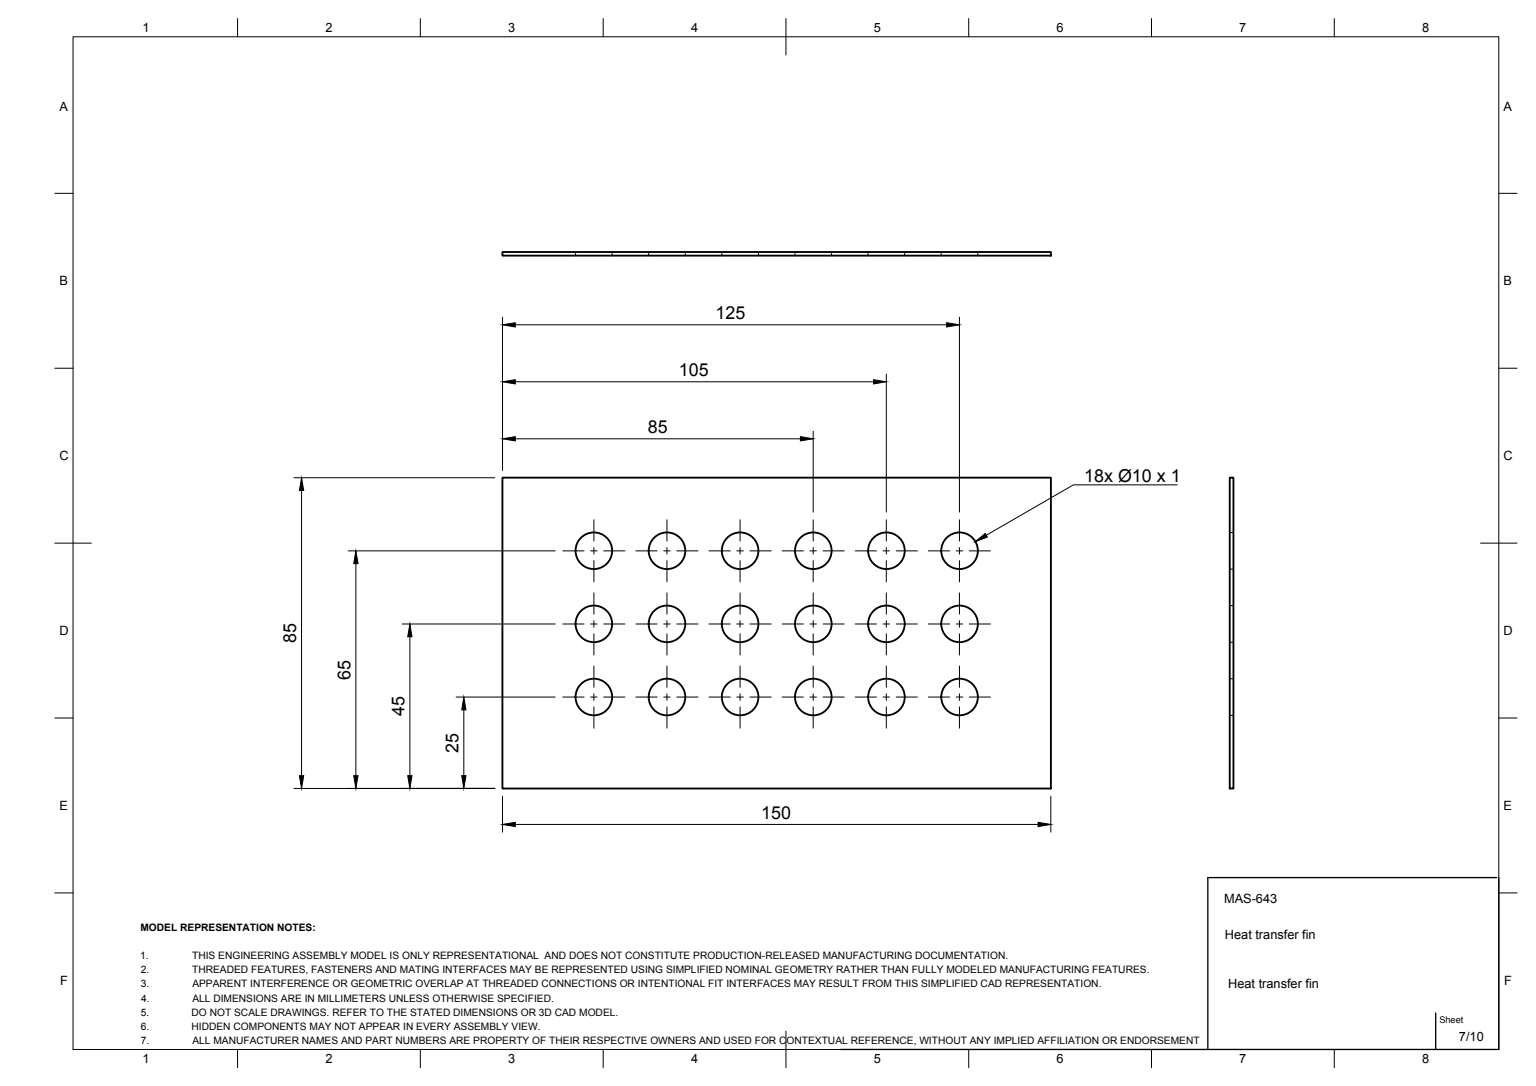
ISO-10303-21;
HEADER;
/* Generated by software containing ST-Developer
 * from STEP Tools, Inc. (www.steptools.com) 
 */

FILE_DESCRIPTION(
/* description */ ('Independent eighteen-tube parallel-flow evaporator geometry. Repeated
 machined headers and gasketed service covers, eighteen copper tubes, 
twenty-nine punched fins, threaded hose connections and bolted mountin
g feet. Native editable features and instanced parts. Braze details, w
orking fluid, pressure and thermal ratings require engineering selecti
on.'),
/* implementation_level */ '2;1');

FILE_NAME(
/* name */ 'Heat transfer fin.step',
/* time_stamp */ '2026-11-08T20:53:59-08:00',
/* author */ (''),
/* organization */ (''),
/* preprocessor_version */ 'ST-DEVELOPER v20.2',
/* originating_system */ 'Autodesk Translation Framework v15.17.0.0',
/* authorisation */ '');

FILE_SCHEMA (('AUTOMOTIVE_DESIGN { 1 0 10303 214 3 1 1 }'));
ENDSEC;

DATA;
#10=MECHANICAL_DESIGN_GEOMETRIC_PRESENTATION_REPRESENTATION('',(#337),#42620);
#317=SHAPE_REPRESENTATION_RELATIONSHIP('SRR','None',#42727,#327);
#327=ADVANCED_BREP_SHAPE_REPRESENTATION('',(#347),#42614);
#337=STYLED_ITEM('',(#42786),#347);
#347=MANIFOLD_SOLID_BREP('Body1',#10387);
#421=FACE_BOUND('',#1613,.T.);
#422=FACE_BOUND('',#1614,.T.);
#423=FACE_BOUND('',#1615,.T.);
#424=FACE_BOUND('',#1616,.T.);
#425=FACE_BOUND('',#1617,.T.);
#426=FACE_BOUND('',#1618,.T.);
#427=FACE_BOUND('',#1619,.T.);
#428=FACE_BOUND('',#1620,.T.);
#429=FACE_BOUND('',#1621,.T.);
#430=FACE_BOUND('',#1622,.T.);
#431=FACE_BOUND('',#1623,.T.);
#432=FACE_BOUND('',#1624,.T.);
#433=FACE_BOUND('',#1625,.T.);
#434=FACE_BOUND('',#1626,.T.);
#435=FACE_BOUND('',#1627,.T.);
#436=FACE_BOUND('',#1628,.T.);
#437=FACE_BOUND('',#1629,.T.);
#438=FACE_BOUND('',#1630,.T.);
#439=FACE_BOUND('',#1632,.T.);
#440=FACE_BOUND('',#1633,.T.);
#441=FACE_BOUND('',#1634,.T.);
#442=FACE_BOUND('',#1635,.T.);
#443=FACE_BOUND('',#1636,.T.);
#444=FACE_BOUND('',#1637,.T.);
#445=FACE_BOUND('',#1638,.T.);
#446=FACE_BOUND('',#1639,.T.);
#447=FACE_BOUND('',#1640,.T.);
#448=FACE_BOUND('',#1641,.T.);
#449=FACE_BOUND('',#1642,.T.);
#450=FACE_BOUND('',#1643,.T.);
#451=FACE_BOUND('',#1644,.T.);
#452=FACE_BOUND('',#1645,.T.);
#453=FACE_BOUND('',#1646,.T.);
#454=FACE_BOUND('',#1647,.T.);
#455=FACE_BOUND('',#1648,.T.);
#456=FACE_BOUND('',#1649,.T.);
#535=PLANE('',#11027);
#536=PLANE('',#11028);
#537=PLANE('',#11029);
#538=PLANE('',#11030);
#539=PLANE('',#11031);
#540=PLANE('',#11032);
#978=FACE_OUTER_BOUND('',#1590,.T.);
#979=FACE_OUTER_BOUND('',#1591,.T.);
#980=FACE_OUTER_BOUND('',#1592,.T.);
#981=FACE_OUTER_BOUND('',#1593,.T.);
#982=FACE_OUTER_BOUND('',#1594,.T.);
#983=FACE_OUTER_BOUND('',#1595,.T.);
#984=FACE_OUTER_BOUND('',#1596,.T.);
#985=FACE_OUTER_BOUND('',#1597,.T.);
#986=FACE_OUTER_BOUND('',#1598,.T.);
#987=FACE_OUTER_BOUND('',#1599,.T.);
#988=FACE_OUTER_BOUND('',#1600,.T.);
#989=FACE_OUTER_BOUND('',#1601,.T.);
#990=FACE_OUTER_BOUND('',#1602,.T.);
#991=FACE_OUTER_BOUND('',#1603,.T.);
#992=FACE_OUTER_BOUND('',#1604,.T.);
#993=FACE_OUTER_BOUND('',#1605,.T.);
#994=FACE_OUTER_BOUND('',#1606,.T.);
#995=FACE_OUTER_BOUND('',#1607,.T.);
#996=FACE_OUTER_BOUND('',#1608,.T.);
#997=FACE_OUTER_BOUND('',#1609,.T.);
#998=FACE_OUTER_BOUND('',#1610,.T.);
#999=FACE_OUTER_BOUND('',#1611,.T.);
#1000=FACE_OUTER_BOUND('',#1612,.T.);
#1001=FACE_OUTER_BOUND('',#1631,.T.);
#1590=EDGE_LOOP('',(#8543,#8544,#8545,#8546));
#1591=EDGE_LOOP('',(#8547,#8548,#8549,#8550));
#1592=EDGE_LOOP('',(#8551,#8552,#8553,#8554));
#1593=EDGE_LOOP('',(#8555,#8556,#8557,#8558));
#1594=EDGE_LOOP('',(#8559,#8560,#8561,#8562));
#1595=EDGE_LOOP('',(#8563,#8564,#8565,#8566));
#1596=EDGE_LOOP('',(#8567,#8568,#8569,#8570));
#1597=EDGE_LOOP('',(#8571,#8572,#8573,#8574));
#1598=EDGE_LOOP('',(#8575,#8576,#8577,#8578));
#1599=EDGE_LOOP('',(#8579,#8580,#8581,#8582));
#1600=EDGE_LOOP('',(#8583,#8584,#8585,#8586));
#1601=EDGE_LOOP('',(#8587,#8588,#8589,#8590));
#1602=EDGE_LOOP('',(#8591,#8592,#8593,#8594));
#1603=EDGE_LOOP('',(#8595,#8596,#8597,#8598));
#1604=EDGE_LOOP('',(#8599,#8600,#8601,#8602));
#1605=EDGE_LOOP('',(#8603,#8604,#8605,#8606));
#1606=EDGE_LOOP('',(#8607,#8608,#8609,#8610));
#1607=EDGE_LOOP('',(#8611,#8612,#8613,#8614));
#1608=EDGE_LOOP('',(#8615,#8616,#8617,#8618));
#1609=EDGE_LOOP('',(#8619,#8620,#8621,#8622));
#1610=EDGE_LOOP('',(#8623,#8624,#8625,#8626));
#1611=EDGE_LOOP('',(#8627,#8628,#8629,#8630));
#1612=EDGE_LOOP('',(#8631,#8632,#8633,#8634));
#1613=EDGE_LOOP('',(#8635));
#1614=EDGE_LOOP('',(#8636));
#1615=EDGE_LOOP('',(#8637));
#1616=EDGE_LOOP('',(#8638));
#1617=EDGE_LOOP('',(#8639));
#1618=EDGE_LOOP('',(#8640));
#1619=EDGE_LOOP('',(#8641));
#1620=EDGE_LOOP('',(#8642));
#1621=EDGE_LOOP('',(#8643));
#1622=EDGE_LOOP('',(#8644));
#1623=EDGE_LOOP('',(#8645));
#1624=EDGE_LOOP('',(#8646));
#1625=EDGE_LOOP('',(#8647));
#1626=EDGE_LOOP('',(#8648));
#1627=EDGE_LOOP('',(#8649));
#1628=EDGE_LOOP('',(#8650));
#1629=EDGE_LOOP('',(#8651));
#1630=EDGE_LOOP('',(#8652));
#1631=EDGE_LOOP('',(#8653,#8654,#8655,#8656));
#1632=EDGE_LOOP('',(#8657));
#1633=EDGE_LOOP('',(#8658));
#1634=EDGE_LOOP('',(#8659));
#1635=EDGE_LOOP('',(#8660));
#1636=EDGE_LOOP('',(#8661));
#1637=EDGE_LOOP('',(#8662));
#1638=EDGE_LOOP('',(#8663));
#1639=EDGE_LOOP('',(#8664));
#1640=EDGE_LOOP('',(#8665));
#1641=EDGE_LOOP('',(#8666));
#1642=EDGE_LOOP('',(#8667));
#1643=EDGE_LOOP('',(#8668));
#1644=EDGE_LOOP('',(#8669));
#1645=EDGE_LOOP('',(#8670));
#1646=EDGE_LOOP('',(#8671));
#1647=EDGE_LOOP('',(#8672));
#1648=EDGE_LOOP('',(#8673));
#1649=EDGE_LOOP('',(#8674));
#1931=CIRCLE('',#10974,5.);
#1932=CIRCLE('',#10975,5.);
#1933=CIRCLE('',#10977,5.);
#1934=CIRCLE('',#10978,5.);
#1935=CIRCLE('',#10980,5.);
#1936=CIRCLE('',#10981,5.);
#1937=CIRCLE('',#10983,5.);
#1938=CIRCLE('',#10984,5.);
#1939=CIRCLE('',#10986,5.);
#1940=CIRCLE('',#10987,5.);
#1941=CIRCLE('',#10989,5.);
#1942=CIRCLE('',#10990,5.);
#1943=CIRCLE('',#10992,5.);
#1944=CIRCLE('',#10993,5.);
#1945=CIRCLE('',#10995,5.);
#1946=CIRCLE('',#10996,5.);
#1947=CIRCLE('',#10998,5.);
#1948=CIRCLE('',#10999,5.);
#1949=CIRCLE('',#11001,5.);
#1950=CIRCLE('',#11002,5.);
#1951=CIRCLE('',#11004,5.);
#1952=CIRCLE('',#11005,5.);
#1953=CIRCLE('',#11007,5.);
#1954=CIRCLE('',#11008,5.);
#1955=CIRCLE('',#11010,5.);
#1956=CIRCLE('',#11011,5.);
#1957=CIRCLE('',#11013,5.);
#1958=CIRCLE('',#11014,5.);
#1959=CIRCLE('',#11016,5.);
#1960=CIRCLE('',#11017,5.);
#1961=CIRCLE('',#11019,5.);
#1962=CIRCLE('',#11020,5.);
#1963=CIRCLE('',#11022,5.);
#1964=CIRCLE('',#11023,5.);
#1965=CIRCLE('',#11025,5.);
#1966=CIRCLE('',#11026,5.);
#3164=LINE('',#34984,#3702);
#3165=LINE('',#34990,#3703);
#3166=LINE('',#34996,#3704);
#3167=LINE('',#35002,#3705);
#3168=LINE('',#35008,#3706);
#3169=LINE('',#35014,#3707);
#3170=LINE('',#35020,#3708);
#3171=LINE('',#35026,#3709);
#3172=LINE('',#35032,#3710);
#3173=LINE('',#35038,#3711);
#3174=LINE('',#35044,#3712);
#3175=LINE('',#35050,#3713);
#3176=LINE('',#35056,#3714);
#3177=LINE('',#35062,#3715);
#3178=LINE('',#35068,#3716);
#3179=LINE('',#35074,#3717);
#3180=LINE('',#35080,#3718);
#3181=LINE('',#35086,#3719);
#3182=LINE('',#35091,#3720);
#3183=LINE('',#35093,#3721);
#3184=LINE('',#35095,#3722);
#3185=LINE('',#35096,#3723);
#3186=LINE('',#35099,#3724);
#3187=LINE('',#35101,#3725);
#3188=LINE('',#35102,#3726);
#3189=LINE('',#35105,#3727);
#3190=LINE('',#35107,#3728);
#3191=LINE('',#35108,#3729);
#3192=LINE('',#35110,#3730);
#3193=LINE('',#35111,#3731);
#3702=VECTOR('',#12613,5.);
#3703=VECTOR('',#12620,5.);
#3704=VECTOR('',#12627,5.);
#3705=VECTOR('',#12634,5.);
#3706=VECTOR('',#12641,5.);
#3707=VECTOR('',#12648,5.);
#3708=VECTOR('',#12655,5.);
#3709=VECTOR('',#12662,5.);
#3710=VECTOR('',#12669,5.);
#3711=VECTOR('',#12676,5.);
#3712=VECTOR('',#12683,5.);
#3713=VECTOR('',#12690,5.);
#3714=VECTOR('',#12697,5.);
#3715=VECTOR('',#12704,5.);
#3716=VECTOR('',#12711,5.);
#3717=VECTOR('',#12718,5.);
#3718=VECTOR('',#12725,5.);
#3719=VECTOR('',#12732,5.);
#3720=VECTOR('',#12737,10.);
#3721=VECTOR('',#12738,10.);
#3722=VECTOR('',#12739,10.);
#3723=VECTOR('',#12740,10.);
#3724=VECTOR('',#12743,10.);
#3725=VECTOR('',#12744,10.);
#3726=VECTOR('',#12745,10.);
#3727=VECTOR('',#12748,10.);
#3728=VECTOR('',#12749,10.);
#3729=VECTOR('',#12750,10.);
#3730=VECTOR('',#12753,10.);
#3731=VECTOR('',#12754,10.);
#4587=VERTEX_POINT('',#34981);
#4588=VERTEX_POINT('',#34983);
#4589=VERTEX_POINT('',#34987);
#4590=VERTEX_POINT('',#34989);
#4591=VERTEX_POINT('',#34993);
#4592=VERTEX_POINT('',#34995);
#4593=VERTEX_POINT('',#34999);
#4594=VERTEX_POINT('',#35001);
#4595=VERTEX_POINT('',#35005);
#4596=VERTEX_POINT('',#35007);
#4597=VERTEX_POINT('',#35011);
#4598=VERTEX_POINT('',#35013);
#4599=VERTEX_POINT('',#35017);
#4600=VERTEX_POINT('',#35019);
#4601=VERTEX_POINT('',#35023);
#4602=VERTEX_POINT('',#35025);
#4603=VERTEX_POINT('',#35029);
#4604=VERTEX_POINT('',#35031);
#4605=VERTEX_POINT('',#35035);
#4606=VERTEX_POINT('',#35037);
#4607=VERTEX_POINT('',#35041);
#4608=VERTEX_POINT('',#35043);
#4609=VERTEX_POINT('',#35047);
#4610=VERTEX_POINT('',#35049);
#4611=VERTEX_POINT('',#35053);
#4612=VERTEX_POINT('',#35055);
#4613=VERTEX_POINT('',#35059);
#4614=VERTEX_POINT('',#35061);
#4615=VERTEX_POINT('',#35065);
#4616=VERTEX_POINT('',#35067);
#4617=VERTEX_POINT('',#35071);
#4618=VERTEX_POINT('',#35073);
#4619=VERTEX_POINT('',#35077);
#4620=VERTEX_POINT('',#35079);
#4621=VERTEX_POINT('',#35083);
#4622=VERTEX_POINT('',#35085);
#4623=VERTEX_POINT('',#35089);
#4624=VERTEX_POINT('',#35090);
#4625=VERTEX_POINT('',#35092);
#4626=VERTEX_POINT('',#35094);
#4627=VERTEX_POINT('',#35098);
#4628=VERTEX_POINT('',#35100);
#4629=VERTEX_POINT('',#35104);
#4630=VERTEX_POINT('',#35106);
#5954=EDGE_CURVE('',#4587,#4587,#1931,.T.);
#5955=EDGE_CURVE('',#4587,#4588,#3164,.T.);
#5956=EDGE_CURVE('',#4588,#4588,#1932,.T.);
#5957=EDGE_CURVE('',#4589,#4589,#1933,.T.);
#5958=EDGE_CURVE('',#4589,#4590,#3165,.T.);
#5959=EDGE_CURVE('',#4590,#4590,#1934,.T.);
#5960=EDGE_CURVE('',#4591,#4591,#1935,.T.);
#5961=EDGE_CURVE('',#4591,#4592,#3166,.T.);
#5962=EDGE_CURVE('',#4592,#4592,#1936,.T.);
#5963=EDGE_CURVE('',#4593,#4593,#1937,.T.);
#5964=EDGE_CURVE('',#4593,#4594,#3167,.T.);
#5965=EDGE_CURVE('',#4594,#4594,#1938,.T.);
#5966=EDGE_CURVE('',#4595,#4595,#1939,.T.);
#5967=EDGE_CURVE('',#4595,#4596,#3168,.T.);
#5968=EDGE_CURVE('',#4596,#4596,#1940,.T.);
#5969=EDGE_CURVE('',#4597,#4597,#1941,.T.);
#5970=EDGE_CURVE('',#4597,#4598,#3169,.T.);
#5971=EDGE_CURVE('',#4598,#4598,#1942,.T.);
#5972=EDGE_CURVE('',#4599,#4599,#1943,.T.);
#5973=EDGE_CURVE('',#4599,#4600,#3170,.T.);
#5974=EDGE_CURVE('',#4600,#4600,#1944,.T.);
#5975=EDGE_CURVE('',#4601,#4601,#1945,.T.);
#5976=EDGE_CURVE('',#4601,#4602,#3171,.T.);
#5977=EDGE_CURVE('',#4602,#4602,#1946,.T.);
#5978=EDGE_CURVE('',#4603,#4603,#1947,.T.);
#5979=EDGE_CURVE('',#4603,#4604,#3172,.T.);
#5980=EDGE_CURVE('',#4604,#4604,#1948,.T.);
#5981=EDGE_CURVE('',#4605,#4605,#1949,.T.);
#5982=EDGE_CURVE('',#4605,#4606,#3173,.T.);
#5983=EDGE_CURVE('',#4606,#4606,#1950,.T.);
#5984=EDGE_CURVE('',#4607,#4607,#1951,.T.);
#5985=EDGE_CURVE('',#4607,#4608,#3174,.T.);
#5986=EDGE_CURVE('',#4608,#4608,#1952,.T.);
#5987=EDGE_CURVE('',#4609,#4609,#1953,.T.);
#5988=EDGE_CURVE('',#4609,#4610,#3175,.T.);
#5989=EDGE_CURVE('',#4610,#4610,#1954,.T.);
#5990=EDGE_CURVE('',#4611,#4611,#1955,.T.);
#5991=EDGE_CURVE('',#4611,#4612,#3176,.T.);
#5992=EDGE_CURVE('',#4612,#4612,#1956,.T.);
#5993=EDGE_CURVE('',#4613,#4613,#1957,.T.);
#5994=EDGE_CURVE('',#4613,#4614,#3177,.T.);
#5995=EDGE_CURVE('',#4614,#4614,#1958,.T.);
#5996=EDGE_CURVE('',#4615,#4615,#1959,.T.);
#5997=EDGE_CURVE('',#4615,#4616,#3178,.T.);
#5998=EDGE_CURVE('',#4616,#4616,#1960,.T.);
#5999=EDGE_CURVE('',#4617,#4617,#1961,.T.);
#6000=EDGE_CURVE('',#4617,#4618,#3179,.T.);
#6001=EDGE_CURVE('',#4618,#4618,#1962,.T.);
#6002=EDGE_CURVE('',#4619,#4619,#1963,.T.);
#6003=EDGE_CURVE('',#4619,#4620,#3180,.T.);
#6004=EDGE_CURVE('',#4620,#4620,#1964,.T.);
#6005=EDGE_CURVE('',#4621,#4621,#1965,.T.);
#6006=EDGE_CURVE('',#4621,#4622,#3181,.T.);
#6007=EDGE_CURVE('',#4622,#4622,#1966,.T.);
#6008=EDGE_CURVE('',#4623,#4624,#3182,.T.);
#6009=EDGE_CURVE('',#4624,#4625,#3183,.F.);
#6010=EDGE_CURVE('',#4626,#4625,#3184,.T.);
#6011=EDGE_CURVE('',#4623,#4626,#3185,.T.);
#6012=EDGE_CURVE('',#4627,#4623,#3186,.F.);
#6013=EDGE_CURVE('',#4628,#4626,#3187,.F.);
#6014=EDGE_CURVE('',#4627,#4628,#3188,.T.);
#6015=EDGE_CURVE('',#4629,#4627,#3189,.F.);
#6016=EDGE_CURVE('',#4630,#4628,#3190,.F.);
#6017=EDGE_CURVE('',#4629,#4630,#3191,.F.);
#6018=EDGE_CURVE('',#4624,#4629,#3192,.F.);
#6019=EDGE_CURVE('',#4625,#4630,#3193,.F.);
#8543=ORIENTED_EDGE('',*,*,#5954,.F.);
#8544=ORIENTED_EDGE('',*,*,#5955,.T.);
#8545=ORIENTED_EDGE('',*,*,#5956,.F.);
#8546=ORIENTED_EDGE('',*,*,#5955,.F.);
#8547=ORIENTED_EDGE('',*,*,#5957,.F.);
#8548=ORIENTED_EDGE('',*,*,#5958,.T.);
#8549=ORIENTED_EDGE('',*,*,#5959,.F.);
#8550=ORIENTED_EDGE('',*,*,#5958,.F.);
#8551=ORIENTED_EDGE('',*,*,#5960,.F.);
#8552=ORIENTED_EDGE('',*,*,#5961,.T.);
#8553=ORIENTED_EDGE('',*,*,#5962,.F.);
#8554=ORIENTED_EDGE('',*,*,#5961,.F.);
#8555=ORIENTED_EDGE('',*,*,#5963,.F.);
#8556=ORIENTED_EDGE('',*,*,#5964,.T.);
#8557=ORIENTED_EDGE('',*,*,#5965,.F.);
#8558=ORIENTED_EDGE('',*,*,#5964,.F.);
#8559=ORIENTED_EDGE('',*,*,#5966,.F.);
#8560=ORIENTED_EDGE('',*,*,#5967,.T.);
#8561=ORIENTED_EDGE('',*,*,#5968,.F.);
#8562=ORIENTED_EDGE('',*,*,#5967,.F.);
#8563=ORIENTED_EDGE('',*,*,#5969,.F.);
#8564=ORIENTED_EDGE('',*,*,#5970,.T.);
#8565=ORIENTED_EDGE('',*,*,#5971,.F.);
#8566=ORIENTED_EDGE('',*,*,#5970,.F.);
#8567=ORIENTED_EDGE('',*,*,#5972,.F.);
#8568=ORIENTED_EDGE('',*,*,#5973,.T.);
#8569=ORIENTED_EDGE('',*,*,#5974,.F.);
#8570=ORIENTED_EDGE('',*,*,#5973,.F.);
#8571=ORIENTED_EDGE('',*,*,#5975,.F.);
#8572=ORIENTED_EDGE('',*,*,#5976,.T.);
#8573=ORIENTED_EDGE('',*,*,#5977,.F.);
#8574=ORIENTED_EDGE('',*,*,#5976,.F.);
#8575=ORIENTED_EDGE('',*,*,#5978,.F.);
#8576=ORIENTED_EDGE('',*,*,#5979,.T.);
#8577=ORIENTED_EDGE('',*,*,#5980,.F.);
#8578=ORIENTED_EDGE('',*,*,#5979,.F.);
#8579=ORIENTED_EDGE('',*,*,#5981,.F.);
#8580=ORIENTED_EDGE('',*,*,#5982,.T.);
#8581=ORIENTED_EDGE('',*,*,#5983,.F.);
#8582=ORIENTED_EDGE('',*,*,#5982,.F.);
#8583=ORIENTED_EDGE('',*,*,#5984,.F.);
#8584=ORIENTED_EDGE('',*,*,#5985,.T.);
#8585=ORIENTED_EDGE('',*,*,#5986,.F.);
#8586=ORIENTED_EDGE('',*,*,#5985,.F.);
#8587=ORIENTED_EDGE('',*,*,#5987,.F.);
#8588=ORIENTED_EDGE('',*,*,#5988,.T.);
#8589=ORIENTED_EDGE('',*,*,#5989,.F.);
#8590=ORIENTED_EDGE('',*,*,#5988,.F.);
#8591=ORIENTED_EDGE('',*,*,#5990,.F.);
#8592=ORIENTED_EDGE('',*,*,#5991,.T.);
#8593=ORIENTED_EDGE('',*,*,#5992,.F.);
#8594=ORIENTED_EDGE('',*,*,#5991,.F.);
#8595=ORIENTED_EDGE('',*,*,#5993,.F.);
#8596=ORIENTED_EDGE('',*,*,#5994,.T.);
#8597=ORIENTED_EDGE('',*,*,#5995,.F.);
#8598=ORIENTED_EDGE('',*,*,#5994,.F.);
#8599=ORIENTED_EDGE('',*,*,#5996,.F.);
#8600=ORIENTED_EDGE('',*,*,#5997,.T.);
#8601=ORIENTED_EDGE('',*,*,#5998,.F.);
#8602=ORIENTED_EDGE('',*,*,#5997,.F.);
#8603=ORIENTED_EDGE('',*,*,#5999,.F.);
#8604=ORIENTED_EDGE('',*,*,#6000,.T.);
#8605=ORIENTED_EDGE('',*,*,#6001,.F.);
#8606=ORIENTED_EDGE('',*,*,#6000,.F.);
#8607=ORIENTED_EDGE('',*,*,#6002,.F.);
#8608=ORIENTED_EDGE('',*,*,#6003,.T.);
#8609=ORIENTED_EDGE('',*,*,#6004,.F.);
#8610=ORIENTED_EDGE('',*,*,#6003,.F.);
#8611=ORIENTED_EDGE('',*,*,#6005,.F.);
#8612=ORIENTED_EDGE('',*,*,#6006,.T.);
#8613=ORIENTED_EDGE('',*,*,#6007,.F.);
#8614=ORIENTED_EDGE('',*,*,#6006,.F.);
#8615=ORIENTED_EDGE('',*,*,#6008,.T.);
#8616=ORIENTED_EDGE('',*,*,#6009,.T.);
#8617=ORIENTED_EDGE('',*,*,#6010,.F.);
#8618=ORIENTED_EDGE('',*,*,#6011,.F.);
#8619=ORIENTED_EDGE('',*,*,#6012,.T.);
#8620=ORIENTED_EDGE('',*,*,#6011,.T.);
#8621=ORIENTED_EDGE('',*,*,#6013,.F.);
#8622=ORIENTED_EDGE('',*,*,#6014,.F.);
#8623=ORIENTED_EDGE('',*,*,#6015,.T.);
#8624=ORIENTED_EDGE('',*,*,#6014,.T.);
#8625=ORIENTED_EDGE('',*,*,#6016,.F.);
#8626=ORIENTED_EDGE('',*,*,#6017,.F.);
#8627=ORIENTED_EDGE('',*,*,#6018,.T.);
#8628=ORIENTED_EDGE('',*,*,#6017,.T.);
#8629=ORIENTED_EDGE('',*,*,#6019,.F.);
#8630=ORIENTED_EDGE('',*,*,#6009,.F.);
#8631=ORIENTED_EDGE('',*,*,#6019,.T.);
#8632=ORIENTED_EDGE('',*,*,#6016,.T.);
#8633=ORIENTED_EDGE('',*,*,#6013,.T.);
#8634=ORIENTED_EDGE('',*,*,#6010,.T.);
#8635=ORIENTED_EDGE('',*,*,#6005,.T.);
#8636=ORIENTED_EDGE('',*,*,#6002,.T.);
#8637=ORIENTED_EDGE('',*,*,#5999,.T.);
#8638=ORIENTED_EDGE('',*,*,#5996,.T.);
#8639=ORIENTED_EDGE('',*,*,#5993,.T.);
#8640=ORIENTED_EDGE('',*,*,#5990,.T.);
#8641=ORIENTED_EDGE('',*,*,#5987,.T.);
#8642=ORIENTED_EDGE('',*,*,#5984,.T.);
#8643=ORIENTED_EDGE('',*,*,#5981,.T.);
#8644=ORIENTED_EDGE('',*,*,#5978,.T.);
#8645=ORIENTED_EDGE('',*,*,#5975,.T.);
#8646=ORIENTED_EDGE('',*,*,#5972,.T.);
#8647=ORIENTED_EDGE('',*,*,#5969,.T.);
#8648=ORIENTED_EDGE('',*,*,#5966,.T.);
#8649=ORIENTED_EDGE('',*,*,#5963,.T.);
#8650=ORIENTED_EDGE('',*,*,#5960,.T.);
#8651=ORIENTED_EDGE('',*,*,#5957,.T.);
#8652=ORIENTED_EDGE('',*,*,#5954,.T.);
#8653=ORIENTED_EDGE('',*,*,#6018,.F.);
#8654=ORIENTED_EDGE('',*,*,#6008,.F.);
#8655=ORIENTED_EDGE('',*,*,#6012,.F.);
#8656=ORIENTED_EDGE('',*,*,#6015,.F.);
#8657=ORIENTED_EDGE('',*,*,#6007,.T.);
#8658=ORIENTED_EDGE('',*,*,#6004,.T.);
#8659=ORIENTED_EDGE('',*,*,#6001,.T.);
#8660=ORIENTED_EDGE('',*,*,#5998,.T.);
#8661=ORIENTED_EDGE('',*,*,#5995,.T.);
#8662=ORIENTED_EDGE('',*,*,#5992,.T.);
#8663=ORIENTED_EDGE('',*,*,#5989,.T.);
#8664=ORIENTED_EDGE('',*,*,#5986,.T.);
#8665=ORIENTED_EDGE('',*,*,#5983,.T.);
#8666=ORIENTED_EDGE('',*,*,#5980,.T.);
#8667=ORIENTED_EDGE('',*,*,#5977,.T.);
#8668=ORIENTED_EDGE('',*,*,#5974,.T.);
#8669=ORIENTED_EDGE('',*,*,#5971,.T.);
#8670=ORIENTED_EDGE('',*,*,#5968,.T.);
#8671=ORIENTED_EDGE('',*,*,#5965,.T.);
#8672=ORIENTED_EDGE('',*,*,#5962,.T.);
#8673=ORIENTED_EDGE('',*,*,#5959,.T.);
#8674=ORIENTED_EDGE('',*,*,#5956,.T.);
#9722=CYLINDRICAL_SURFACE('',#10973,5.);
#9723=CYLINDRICAL_SURFACE('',#10976,5.);
#9724=CYLINDRICAL_SURFACE('',#10979,5.);
#9725=CYLINDRICAL_SURFACE('',#10982,5.);
#9726=CYLINDRICAL_SURFACE('',#10985,5.);
#9727=CYLINDRICAL_SURFACE('',#10988,5.);
#9728=CYLINDRICAL_SURFACE('',#10991,5.);
#9729=CYLINDRICAL_SURFACE('',#10994,5.);
#9730=CYLINDRICAL_SURFACE('',#10997,5.);
#9731=CYLINDRICAL_SURFACE('',#11000,5.);
#9732=CYLINDRICAL_SURFACE('',#11003,5.);
#9733=CYLINDRICAL_SURFACE('',#11006,5.);
#9734=CYLINDRICAL_SURFACE('',#11009,5.);
#9735=CYLINDRICAL_SURFACE('',#11012,5.);
#9736=CYLINDRICAL_SURFACE('',#11015,5.);
#9737=CYLINDRICAL_SURFACE('',#11018,5.);
#9738=CYLINDRICAL_SURFACE('',#11021,5.);
#9739=CYLINDRICAL_SURFACE('',#11024,5.);
#10214=ADVANCED_FACE('',(#978),#9722,.F.);
#10215=ADVANCED_FACE('',(#979),#9723,.F.);
#10216=ADVANCED_FACE('',(#980),#9724,.F.);
#10217=ADVANCED_FACE('',(#981),#9725,.F.);
#10218=ADVANCED_FACE('',(#982),#9726,.F.);
#10219=ADVANCED_FACE('',(#983),#9727,.F.);
#10220=ADVANCED_FACE('',(#984),#9728,.F.);
#10221=ADVANCED_FACE('',(#985),#9729,.F.);
#10222=ADVANCED_FACE('',(#986),#9730,.F.);
#10223=ADVANCED_FACE('',(#987),#9731,.F.);
#10224=ADVANCED_FACE('',(#988),#9732,.F.);
#10225=ADVANCED_FACE('',(#989),#9733,.F.);
#10226=ADVANCED_FACE('',(#990),#9734,.F.);
#10227=ADVANCED_FACE('',(#991),#9735,.F.);
#10228=ADVANCED_FACE('',(#992),#9736,.F.);
#10229=ADVANCED_FACE('',(#993),#9737,.F.);
#10230=ADVANCED_FACE('',(#994),#9738,.F.);
#10231=ADVANCED_FACE('',(#995),#9739,.F.);
#10232=ADVANCED_FACE('',(#996),#535,.T.);
#10233=ADVANCED_FACE('',(#997),#536,.T.);
#10234=ADVANCED_FACE('',(#998),#537,.T.);
#10235=ADVANCED_FACE('',(#999),#538,.T.);
#10236=ADVANCED_FACE('',(#1000,#421,#422,#423,#424,#425,#426,#427,#428,
#429,#430,#431,#432,#433,#434,#435,#436,#437,#438),#539,.T.);
#10237=ADVANCED_FACE('',(#1001,#439,#440,#441,#442,#443,#444,#445,#446,
#447,#448,#449,#450,#451,#452,#453,#454,#455,#456),#540,.F.);
#10387=CLOSED_SHELL('',(#10214,#10215,#10216,#10217,#10218,#10219,#10220,
#10221,#10222,#10223,#10224,#10225,#10226,#10227,#10228,#10229,#10230,#10231,
#10232,#10233,#10234,#10235,#10236,#10237));
#10972=AXIS2_PLACEMENT_3D('',#34979,#12607,#12608);
#10973=AXIS2_PLACEMENT_3D('',#34980,#12609,#12610);
#10974=AXIS2_PLACEMENT_3D('',#34982,#12611,#12612);
#10975=AXIS2_PLACEMENT_3D('',#34985,#12614,#12615);
#10976=AXIS2_PLACEMENT_3D('',#34986,#12616,#12617);
#10977=AXIS2_PLACEMENT_3D('',#34988,#12618,#12619);
#10978=AXIS2_PLACEMENT_3D('',#34991,#12621,#12622);
#10979=AXIS2_PLACEMENT_3D('',#34992,#12623,#12624);
#10980=AXIS2_PLACEMENT_3D('',#34994,#12625,#12626);
#10981=AXIS2_PLACEMENT_3D('',#34997,#12628,#12629);
#10982=AXIS2_PLACEMENT_3D('',#34998,#12630,#12631);
#10983=AXIS2_PLACEMENT_3D('',#35000,#12632,#12633);
#10984=AXIS2_PLACEMENT_3D('',#35003,#12635,#12636);
#10985=AXIS2_PLACEMENT_3D('',#35004,#12637,#12638);
#10986=AXIS2_PLACEMENT_3D('',#35006,#12639,#12640);
#10987=AXIS2_PLACEMENT_3D('',#35009,#12642,#12643);
#10988=AXIS2_PLACEMENT_3D('',#35010,#12644,#12645);
#10989=AXIS2_PLACEMENT_3D('',#35012,#12646,#12647);
#10990=AXIS2_PLACEMENT_3D('',#35015,#12649,#12650);
#10991=AXIS2_PLACEMENT_3D('',#35016,#12651,#12652);
#10992=AXIS2_PLACEMENT_3D('',#35018,#12653,#12654);
#10993=AXIS2_PLACEMENT_3D('',#35021,#12656,#12657);
#10994=AXIS2_PLACEMENT_3D('',#35022,#12658,#12659);
#10995=AXIS2_PLACEMENT_3D('',#35024,#12660,#12661);
#10996=AXIS2_PLACEMENT_3D('',#35027,#12663,#12664);
#10997=AXIS2_PLACEMENT_3D('',#35028,#12665,#12666);
#10998=AXIS2_PLACEMENT_3D('',#35030,#12667,#12668);
#10999=AXIS2_PLACEMENT_3D('',#35033,#12670,#12671);
#11000=AXIS2_PLACEMENT_3D('',#35034,#12672,#12673);
#11001=AXIS2_PLACEMENT_3D('',#35036,#12674,#12675);
#11002=AXIS2_PLACEMENT_3D('',#35039,#12677,#12678);
#11003=AXIS2_PLACEMENT_3D('',#35040,#12679,#12680);
#11004=AXIS2_PLACEMENT_3D('',#35042,#12681,#12682);
#11005=AXIS2_PLACEMENT_3D('',#35045,#12684,#12685);
#11006=AXIS2_PLACEMENT_3D('',#35046,#12686,#12687);
#11007=AXIS2_PLACEMENT_3D('',#35048,#12688,#12689);
#11008=AXIS2_PLACEMENT_3D('',#35051,#12691,#12692);
#11009=AXIS2_PLACEMENT_3D('',#35052,#12693,#12694);
#11010=AXIS2_PLACEMENT_3D('',#35054,#12695,#12696);
#11011=AXIS2_PLACEMENT_3D('',#35057,#12698,#12699);
#11012=AXIS2_PLACEMENT_3D('',#35058,#12700,#12701);
#11013=AXIS2_PLACEMENT_3D('',#35060,#12702,#12703);
#11014=AXIS2_PLACEMENT_3D('',#35063,#12705,#12706);
#11015=AXIS2_PLACEMENT_3D('',#35064,#12707,#12708);
#11016=AXIS2_PLACEMENT_3D('',#35066,#12709,#12710);
#11017=AXIS2_PLACEMENT_3D('',#35069,#12712,#12713);
#11018=AXIS2_PLACEMENT_3D('',#35070,#12714,#12715);
#11019=AXIS2_PLACEMENT_3D('',#35072,#12716,#12717);
#11020=AXIS2_PLACEMENT_3D('',#35075,#12719,#12720);
#11021=AXIS2_PLACEMENT_3D('',#35076,#12721,#12722);
#11022=AXIS2_PLACEMENT_3D('',#35078,#12723,#12724);
#11023=AXIS2_PLACEMENT_3D('',#35081,#12726,#12727);
#11024=AXIS2_PLACEMENT_3D('',#35082,#12728,#12729);
#11025=AXIS2_PLACEMENT_3D('',#35084,#12730,#12731);
#11026=AXIS2_PLACEMENT_3D('',#35087,#12733,#12734);
#11027=AXIS2_PLACEMENT_3D('',#35088,#12735,#12736);
#11028=AXIS2_PLACEMENT_3D('',#35097,#12741,#12742);
#11029=AXIS2_PLACEMENT_3D('',#35103,#12746,#12747);
#11030=AXIS2_PLACEMENT_3D('',#35109,#12751,#12752);
#11031=AXIS2_PLACEMENT_3D('',#35112,#12755,#12756);
#11032=AXIS2_PLACEMENT_3D('',#35113,#12757,#12758);
#12607=DIRECTION('axis',(0.,0.,1.));
#12608=DIRECTION('refdir',(1.,0.,0.));
#12609=DIRECTION('center_axis',(0.,0.,-1.));
#12610=DIRECTION('ref_axis',(1.,0.,0.));
#12611=DIRECTION('center_axis',(0.,0.,-1.));
#12612=DIRECTION('ref_axis',(1.,0.,0.));
#12613=DIRECTION('',(0.,0.,-1.));
#12614=DIRECTION('center_axis',(0.,0.,1.));
#12615=DIRECTION('ref_axis',(1.,0.,0.));
#12616=DIRECTION('center_axis',(0.,0.,-1.));
#12617=DIRECTION('ref_axis',(1.,0.,0.));
#12618=DIRECTION('center_axis',(0.,0.,-1.));
#12619=DIRECTION('ref_axis',(1.,0.,0.));
#12620=DIRECTION('',(0.,0.,-1.));
#12621=DIRECTION('center_axis',(0.,0.,1.));
#12622=DIRECTION('ref_axis',(1.,0.,0.));
#12623=DIRECTION('center_axis',(0.,0.,-1.));
#12624=DIRECTION('ref_axis',(1.,0.,0.));
#12625=DIRECTION('center_axis',(0.,0.,-1.));
#12626=DIRECTION('ref_axis',(1.,0.,0.));
#12627=DIRECTION('',(0.,0.,-1.));
#12628=DIRECTION('center_axis',(0.,0.,1.));
#12629=DIRECTION('ref_axis',(1.,0.,0.));
#12630=DIRECTION('center_axis',(0.,0.,-1.));
#12631=DIRECTION('ref_axis',(1.,0.,0.));
#12632=DIRECTION('center_axis',(0.,0.,-1.));
#12633=DIRECTION('ref_axis',(1.,0.,0.));
#12634=DIRECTION('',(0.,0.,-1.));
#12635=DIRECTION('center_axis',(0.,0.,1.));
#12636=DIRECTION('ref_axis',(1.,0.,0.));
#12637=DIRECTION('center_axis',(0.,0.,-1.));
#12638=DIRECTION('ref_axis',(1.,0.,0.));
#12639=DIRECTION('center_axis',(0.,0.,-1.));
#12640=DIRECTION('ref_axis',(1.,0.,0.));
#12641=DIRECTION('',(0.,0.,-1.));
#12642=DIRECTION('center_axis',(0.,0.,1.));
#12643=DIRECTION('ref_axis',(1.,0.,0.));
#12644=DIRECTION('center_axis',(0.,0.,-1.));
#12645=DIRECTION('ref_axis',(1.,0.,0.));
#12646=DIRECTION('center_axis',(0.,0.,-1.));
#12647=DIRECTION('ref_axis',(1.,0.,0.));
#12648=DIRECTION('',(0.,0.,-1.));
#12649=DIRECTION('center_axis',(0.,0.,1.));
#12650=DIRECTION('ref_axis',(1.,0.,0.));
#12651=DIRECTION('center_axis',(0.,0.,-1.));
#12652=DIRECTION('ref_axis',(1.,0.,0.));
#12653=DIRECTION('center_axis',(0.,0.,-1.));
#12654=DIRECTION('ref_axis',(1.,0.,0.));
#12655=DIRECTION('',(0.,0.,-1.));
#12656=DIRECTION('center_axis',(0.,0.,1.));
#12657=DIRECTION('ref_axis',(1.,0.,0.));
#12658=DIRECTION('center_axis',(0.,0.,-1.));
#12659=DIRECTION('ref_axis',(1.,0.,0.));
#12660=DIRECTION('center_axis',(0.,0.,-1.));
#12661=DIRECTION('ref_axis',(1.,0.,0.));
#12662=DIRECTION('',(0.,0.,-1.));
#12663=DIRECTION('center_axis',(0.,0.,1.));
#12664=DIRECTION('ref_axis',(1.,0.,0.));
#12665=DIRECTION('center_axis',(0.,0.,-1.));
#12666=DIRECTION('ref_axis',(1.,0.,0.));
#12667=DIRECTION('center_axis',(0.,0.,-1.));
#12668=DIRECTION('ref_axis',(1.,0.,0.));
#12669=DIRECTION('',(0.,0.,-1.));
#12670=DIRECTION('center_axis',(0.,0.,1.));
#12671=DIRECTION('ref_axis',(1.,0.,0.));
#12672=DIRECTION('center_axis',(0.,0.,-1.));
#12673=DIRECTION('ref_axis',(1.,0.,0.));
#12674=DIRECTION('center_axis',(0.,0.,-1.));
#12675=DIRECTION('ref_axis',(1.,0.,0.));
#12676=DIRECTION('',(0.,0.,-1.));
#12677=DIRECTION('center_axis',(0.,0.,1.));
#12678=DIRECTION('ref_axis',(1.,0.,0.));
#12679=DIRECTION('center_axis',(0.,0.,-1.));
#12680=DIRECTION('ref_axis',(1.,0.,0.));
#12681=DIRECTION('center_axis',(0.,0.,-1.));
#12682=DIRECTION('ref_axis',(1.,0.,0.));
#12683=DIRECTION('',(0.,0.,-1.));
#12684=DIRECTION('center_axis',(0.,0.,1.));
#12685=DIRECTION('ref_axis',(1.,0.,0.));
#12686=DIRECTION('center_axis',(0.,0.,-1.));
#12687=DIRECTION('ref_axis',(1.,0.,0.));
#12688=DIRECTION('center_axis',(0.,0.,-1.));
#12689=DIRECTION('ref_axis',(1.,0.,0.));
#12690=DIRECTION('',(0.,0.,-1.));
#12691=DIRECTION('center_axis',(0.,0.,1.));
#12692=DIRECTION('ref_axis',(1.,0.,0.));
#12693=DIRECTION('center_axis',(0.,0.,-1.));
#12694=DIRECTION('ref_axis',(1.,0.,0.));
#12695=DIRECTION('center_axis',(0.,0.,-1.));
#12696=DIRECTION('ref_axis',(1.,0.,0.));
#12697=DIRECTION('',(0.,0.,-1.));
#12698=DIRECTION('center_axis',(0.,0.,1.));
#12699=DIRECTION('ref_axis',(1.,0.,0.));
#12700=DIRECTION('center_axis',(0.,0.,-1.));
#12701=DIRECTION('ref_axis',(1.,0.,0.));
#12702=DIRECTION('center_axis',(0.,0.,-1.));
#12703=DIRECTION('ref_axis',(1.,0.,0.));
#12704=DIRECTION('',(0.,0.,-1.));
#12705=DIRECTION('center_axis',(0.,0.,1.));
#12706=DIRECTION('ref_axis',(1.,0.,0.));
#12707=DIRECTION('center_axis',(0.,0.,-1.));
#12708=DIRECTION('ref_axis',(1.,0.,0.));
#12709=DIRECTION('center_axis',(0.,0.,-1.));
#12710=DIRECTION('ref_axis',(1.,0.,0.));
#12711=DIRECTION('',(0.,0.,-1.));
#12712=DIRECTION('center_axis',(0.,0.,1.));
#12713=DIRECTION('ref_axis',(1.,0.,0.));
#12714=DIRECTION('center_axis',(0.,0.,-1.));
#12715=DIRECTION('ref_axis',(1.,0.,0.));
#12716=DIRECTION('center_axis',(0.,0.,-1.));
#12717=DIRECTION('ref_axis',(1.,0.,0.));
#12718=DIRECTION('',(0.,0.,-1.));
#12719=DIRECTION('center_axis',(0.,0.,1.));
#12720=DIRECTION('ref_axis',(1.,0.,0.));
#12721=DIRECTION('center_axis',(0.,0.,-1.));
#12722=DIRECTION('ref_axis',(1.,0.,0.));
#12723=DIRECTION('center_axis',(0.,0.,-1.));
#12724=DIRECTION('ref_axis',(1.,0.,0.));
#12725=DIRECTION('',(0.,0.,-1.));
#12726=DIRECTION('center_axis',(0.,0.,1.));
#12727=DIRECTION('ref_axis',(1.,0.,0.));
#12728=DIRECTION('center_axis',(0.,0.,-1.));
#12729=DIRECTION('ref_axis',(1.,0.,0.));
#12730=DIRECTION('center_axis',(0.,0.,-1.));
#12731=DIRECTION('ref_axis',(1.,0.,0.));
#12732=DIRECTION('',(0.,0.,-1.));
#12733=DIRECTION('center_axis',(0.,0.,1.));
#12734=DIRECTION('ref_axis',(1.,0.,0.));
#12735=DIRECTION('center_axis',(0.,1.,0.));
#12736=DIRECTION('ref_axis',(-1.,0.,0.));
#12737=DIRECTION('',(-1.,0.,0.));
#12738=DIRECTION('',(0.,0.,-1.));
#12739=DIRECTION('',(-1.,0.,0.));
#12740=DIRECTION('',(0.,0.,1.));
#12741=DIRECTION('center_axis',(1.,0.,0.));
#12742=DIRECTION('ref_axis',(0.,1.,0.));
#12743=DIRECTION('',(0.,-1.,0.));
#12744=DIRECTION('',(0.,-1.,0.));
#12745=DIRECTION('',(0.,0.,1.));
#12746=DIRECTION('center_axis',(0.,-1.,0.));
#12747=DIRECTION('ref_axis',(1.,0.,0.));
#12748=DIRECTION('',(-1.,0.,0.));
#12749=DIRECTION('',(-1.,0.,0.));
#12750=DIRECTION('',(0.,0.,-1.));
#12751=DIRECTION('center_axis',(-1.,0.,0.));
#12752=DIRECTION('ref_axis',(0.,-1.,0.));
#12753=DIRECTION('',(0.,1.,0.));
#12754=DIRECTION('',(0.,1.,0.));
#12755=DIRECTION('center_axis',(0.,0.,1.));
#12756=DIRECTION('ref_axis',(1.,0.,0.));
#12757=DIRECTION('center_axis',(0.,0.,1.));
#12758=DIRECTION('ref_axis',(1.,0.,0.));
#34979=CARTESIAN_POINT('',(0.,0.,0.));
#34980=CARTESIAN_POINT('Origin',(50.,0.,0.5));
#34981=CARTESIAN_POINT('',(45.,6.12323399573677E-16,1.));
#34982=CARTESIAN_POINT('Origin',(50.,0.,1.));
#34983=CARTESIAN_POINT('',(45.,6.12323399573677E-16,0.));
#34984=CARTESIAN_POINT('',(45.,6.12323399573677E-16,0.5));
#34985=CARTESIAN_POINT('Origin',(50.,0.,0.));
#34986=CARTESIAN_POINT('Origin',(30.,20.,0.5));
#34987=CARTESIAN_POINT('',(25.,20.,1.));
#34988=CARTESIAN_POINT('Origin',(30.,20.,1.));
#34989=CARTESIAN_POINT('',(25.,20.,0.));
#34990=CARTESIAN_POINT('',(25.,20.,0.5));
#34991=CARTESIAN_POINT('Origin',(30.,20.,0.));
#34992=CARTESIAN_POINT('Origin',(30.,-20.,0.5));
#34993=CARTESIAN_POINT('',(25.,-20.,1.));
#34994=CARTESIAN_POINT('Origin',(30.,-20.,1.));
#34995=CARTESIAN_POINT('',(25.,-20.,0.));
#34996=CARTESIAN_POINT('',(25.,-20.,0.5));
#34997=CARTESIAN_POINT('Origin',(30.,-20.,0.));
#34998=CARTESIAN_POINT('Origin',(10.,0.,0.5));
#34999=CARTESIAN_POINT('',(5.,6.12323399573677E-16,1.));
#35000=CARTESIAN_POINT('Origin',(10.,0.,1.));
#35001=CARTESIAN_POINT('',(5.,6.12323399573677E-16,0.));
#35002=CARTESIAN_POINT('',(5.,6.12323399573677E-16,0.5));
#35003=CARTESIAN_POINT('Origin',(10.,0.,0.));
#35004=CARTESIAN_POINT('Origin',(-10.,20.,0.5));
#35005=CARTESIAN_POINT('',(-15.,20.,1.));
#35006=CARTESIAN_POINT('Origin',(-10.,20.,1.));
#35007=CARTESIAN_POINT('',(-15.,20.,0.));
#35008=CARTESIAN_POINT('',(-15.,20.,0.5));
#35009=CARTESIAN_POINT('Origin',(-10.,20.,0.));
#35010=CARTESIAN_POINT('Origin',(-10.,-20.,0.5));
#35011=CARTESIAN_POINT('',(-15.,-20.,1.));
#35012=CARTESIAN_POINT('Origin',(-10.,-20.,1.));
#35013=CARTESIAN_POINT('',(-15.,-20.,0.));
#35014=CARTESIAN_POINT('',(-15.,-20.,0.5));
#35015=CARTESIAN_POINT('Origin',(-10.,-20.,0.));
#35016=CARTESIAN_POINT('Origin',(-30.,0.,0.5));
#35017=CARTESIAN_POINT('',(-35.,6.12323399573677E-16,1.));
#35018=CARTESIAN_POINT('Origin',(-30.,0.,1.));
#35019=CARTESIAN_POINT('',(-35.,6.12323399573677E-16,0.));
#35020=CARTESIAN_POINT('',(-35.,6.12323399573677E-16,0.5));
#35021=CARTESIAN_POINT('Origin',(-30.,0.,0.));
#35022=CARTESIAN_POINT('Origin',(-50.,20.,0.5));
#35023=CARTESIAN_POINT('',(-55.,20.,1.));
#35024=CARTESIAN_POINT('Origin',(-50.,20.,1.));
#35025=CARTESIAN_POINT('',(-55.,20.,0.));
#35026=CARTESIAN_POINT('',(-55.,20.,0.5));
#35027=CARTESIAN_POINT('Origin',(-50.,20.,0.));
#35028=CARTESIAN_POINT('Origin',(-50.,-20.,0.5));
#35029=CARTESIAN_POINT('',(-55.,-20.,1.));
#35030=CARTESIAN_POINT('Origin',(-50.,-20.,1.));
#35031=CARTESIAN_POINT('',(-55.,-20.,0.));
#35032=CARTESIAN_POINT('',(-55.,-20.,0.5));
#35033=CARTESIAN_POINT('Origin',(-50.,-20.,0.));
#35034=CARTESIAN_POINT('Origin',(-50.,0.,0.5));
#35035=CARTESIAN_POINT('',(-55.,6.12323399573677E-16,1.));
#35036=CARTESIAN_POINT('Origin',(-50.,0.,1.));
#35037=CARTESIAN_POINT('',(-55.,6.12323399573677E-16,0.));
#35038=CARTESIAN_POINT('',(-55.,6.12323399573677E-16,0.5));
#35039=CARTESIAN_POINT('Origin',(-50.,0.,0.));
#35040=CARTESIAN_POINT('Origin',(-30.,-20.,0.5));
#35041=CARTESIAN_POINT('',(-35.,-20.,1.));
#35042=CARTESIAN_POINT('Origin',(-30.,-20.,1.));
#35043=CARTESIAN_POINT('',(-35.,-20.,0.));
#35044=CARTESIAN_POINT('',(-35.,-20.,0.5));
#35045=CARTESIAN_POINT('Origin',(-30.,-20.,0.));
#35046=CARTESIAN_POINT('Origin',(-30.,20.,0.5));
#35047=CARTESIAN_POINT('',(-35.,20.,1.));
#35048=CARTESIAN_POINT('Origin',(-30.,20.,1.));
#35049=CARTESIAN_POINT('',(-35.,20.,0.));
#35050=CARTESIAN_POINT('',(-35.,20.,0.5));
#35051=CARTESIAN_POINT('Origin',(-30.,20.,0.));
#35052=CARTESIAN_POINT('Origin',(-10.,0.,0.5));
#35053=CARTESIAN_POINT('',(-15.,6.12323399573677E-16,1.));
#35054=CARTESIAN_POINT('Origin',(-10.,0.,1.));
#35055=CARTESIAN_POINT('',(-15.,6.12323399573677E-16,0.));
#35056=CARTESIAN_POINT('',(-15.,6.12323399573677E-16,0.5));
#35057=CARTESIAN_POINT('Origin',(-10.,0.,0.));
#35058=CARTESIAN_POINT('Origin',(10.,-20.,0.5));
#35059=CARTESIAN_POINT('',(5.,-20.,1.));
#35060=CARTESIAN_POINT('Origin',(10.,-20.,1.));
#35061=CARTESIAN_POINT('',(5.,-20.,0.));
#35062=CARTESIAN_POINT('',(5.,-20.,0.5));
#35063=CARTESIAN_POINT('Origin',(10.,-20.,0.));
#35064=CARTESIAN_POINT('Origin',(10.,20.,0.5));
#35065=CARTESIAN_POINT('',(5.,20.,1.));
#35066=CARTESIAN_POINT('Origin',(10.,20.,1.));
#35067=CARTESIAN_POINT('',(5.,20.,0.));
#35068=CARTESIAN_POINT('',(5.,20.,0.5));
#35069=CARTESIAN_POINT('Origin',(10.,20.,0.));
#35070=CARTESIAN_POINT('Origin',(30.,0.,0.5));
#35071=CARTESIAN_POINT('',(25.,6.12323399573677E-16,1.));
#35072=CARTESIAN_POINT('Origin',(30.,0.,1.));
#35073=CARTESIAN_POINT('',(25.,6.12323399573677E-16,0.));
#35074=CARTESIAN_POINT('',(25.,6.12323399573677E-16,0.5));
#35075=CARTESIAN_POINT('Origin',(30.,0.,0.));
#35076=CARTESIAN_POINT('Origin',(50.,-20.,0.5));
#35077=CARTESIAN_POINT('',(45.,-20.,1.));
#35078=CARTESIAN_POINT('Origin',(50.,-20.,1.));
#35079=CARTESIAN_POINT('',(45.,-20.,0.));
#35080=CARTESIAN_POINT('',(45.,-20.,0.5));
#35081=CARTESIAN_POINT('Origin',(50.,-20.,0.));
#35082=CARTESIAN_POINT('Origin',(50.,20.,0.5));
#35083=CARTESIAN_POINT('',(45.,20.,1.));
#35084=CARTESIAN_POINT('Origin',(50.,20.,1.));
#35085=CARTESIAN_POINT('',(45.,20.,0.));
#35086=CARTESIAN_POINT('',(45.,20.,0.5));
#35087=CARTESIAN_POINT('Origin',(50.,20.,0.));
#35088=CARTESIAN_POINT('Origin',(70.,40.,0.));
#35089=CARTESIAN_POINT('',(75.,40.,0.));
#35090=CARTESIAN_POINT('',(-75.,40.,0.));
#35091=CARTESIAN_POINT('',(70.,40.,0.));
#35092=CARTESIAN_POINT('',(-75.,40.,1.));
#35093=CARTESIAN_POINT('',(-75.,40.,0.));
#35094=CARTESIAN_POINT('',(75.,40.,1.));
#35095=CARTESIAN_POINT('',(70.,40.,1.));
#35096=CARTESIAN_POINT('',(75.,40.,0.));
#35097=CARTESIAN_POINT('Origin',(75.,-40.,0.));
#35098=CARTESIAN_POINT('',(75.,-45.,0.));
#35099=CARTESIAN_POINT('',(75.,-20.,0.));
#35100=CARTESIAN_POINT('',(75.,-45.,1.));
#35101=CARTESIAN_POINT('',(75.,-20.,1.));
#35102=CARTESIAN_POINT('',(75.,-45.,0.));
#35103=CARTESIAN_POINT('Origin',(-70.,-45.,0.));
#35104=CARTESIAN_POINT('',(-75.,-45.,0.));
#35105=CARTESIAN_POINT('',(-35.,-45.,0.));
#35106=CARTESIAN_POINT('',(-75.,-45.,1.));
#35107=CARTESIAN_POINT('',(-35.,-45.,1.));
#35108=CARTESIAN_POINT('',(-75.,-45.,0.));
#35109=CARTESIAN_POINT('Origin',(-75.,40.,0.));
#35110=CARTESIAN_POINT('',(-75.,20.,0.));
#35111=CARTESIAN_POINT('',(-75.,20.,1.));
#35112=CARTESIAN_POINT('Origin',(0.,0.,1.));
#35113=CARTESIAN_POINT('Origin',(0.,0.,0.));
#42602=UNCERTAINTY_MEASURE_WITH_UNIT(LENGTH_MEASURE(0.01),#42621,
'DISTANCE_ACCURACY_VALUE',
'Maximum model space distance between geometric entities at asserted c
onnectivities');
#42608=UNCERTAINTY_MEASURE_WITH_UNIT(LENGTH_MEASURE(0.01),#42621,
'DISTANCE_ACCURACY_VALUE',
'Maximum model space distance between geometric entities at asserted c
onnectivities');
#42614=(
GEOMETRIC_REPRESENTATION_CONTEXT(3)
GLOBAL_UNCERTAINTY_ASSIGNED_CONTEXT((#42602))
GLOBAL_UNIT_ASSIGNED_CONTEXT((#42621,#42623,#42624))
REPRESENTATION_CONTEXT('','3D')
);
#42620=(
GEOMETRIC_REPRESENTATION_CONTEXT(3)
GLOBAL_UNCERTAINTY_ASSIGNED_CONTEXT((#42608))
GLOBAL_UNIT_ASSIGNED_CONTEXT((#42621,#42623,#42624))
REPRESENTATION_CONTEXT('','3D')
);
#42621=(
LENGTH_UNIT()
NAMED_UNIT(*)
SI_UNIT(.MILLI.,.METRE.)
);
#42623=(
NAMED_UNIT(*)
PLANE_ANGLE_UNIT()
SI_UNIT($,.RADIAN.)
);
#42624=(
NAMED_UNIT(*)
SI_UNIT($,.STERADIAN.)
SOLID_ANGLE_UNIT()
);
#42630=SHAPE_DEFINITION_REPRESENTATION(#42641,#42727);
#42641=PRODUCT_DEFINITION_SHAPE('',$,#42739);
#42727=SHAPE_REPRESENTATION('',(#10972),#42614);
#42733=PRODUCT_DEFINITION_CONTEXT('part definition',#42768,'design');
#42739=PRODUCT_DEFINITION('Heat transfer fin','Heat transfer fin',#42750,
#42733);
#42750=PRODUCT_DEFINITION_FORMATION('',$,#42775);
#42768=APPLICATION_CONTEXT(
'Core Data for Automotive Mechanical Design Process');
#42769=PRODUCT_CONTEXT('part definition',#42768,'mechanical');
#42775=PRODUCT('Heat transfer fin','Heat transfer fin',$,(#42769));
#42786=PRESENTATION_STYLE_ASSIGNMENT((#42794));
#42794=SURFACE_STYLE_USAGE(.BOTH.,#42802);
#42802=SURFACE_SIDE_STYLE('',(#42810));
#42810=SURFACE_STYLE_FILL_AREA(#42818);
#42818=FILL_AREA_STYLE('Light gray',(#42826));
#42826=FILL_AREA_STYLE_COLOUR('Light gray',#42834);
#42834=COLOUR_RGB('Light gray',0.725490196078431,0.752941176470588,0.792156862745098);
ENDSEC;
END-ISO-10303-21;
